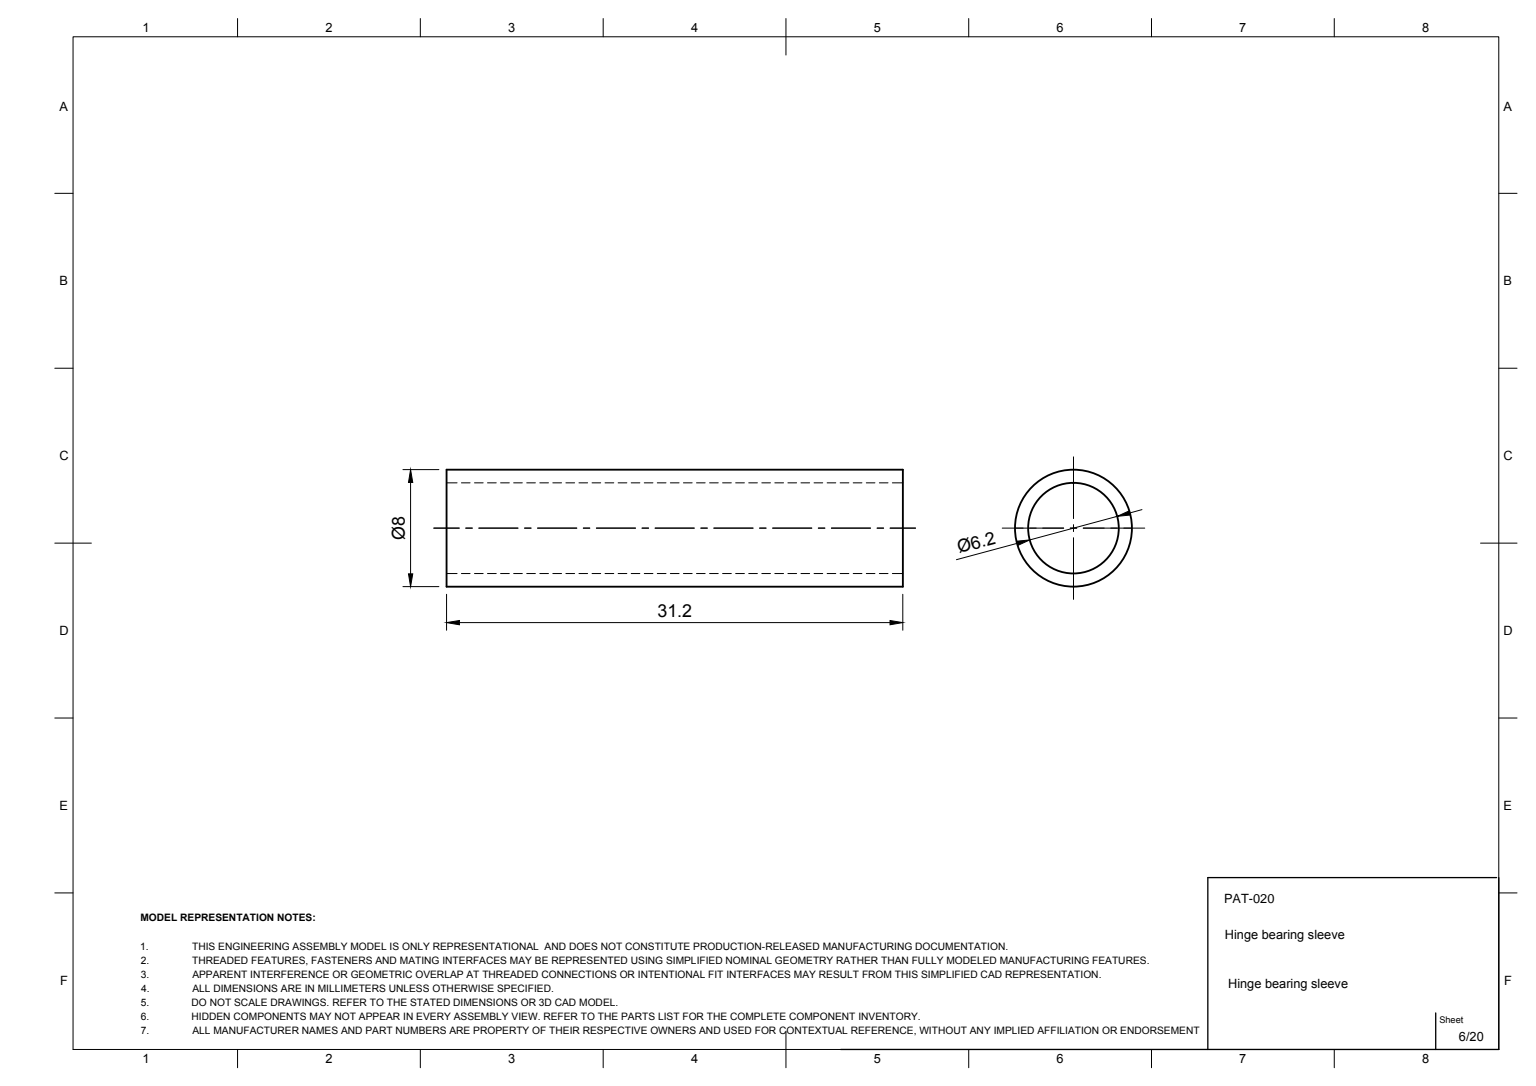
ISO-10303-21;
HEADER;
/* Generated by software containing ST-Developer
 * from STEP Tools, Inc. (www.steptools.com) 
 */

FILE_DESCRIPTION(
/* description */ ('Cable chain and bracket set'),
/* implementation_level */ '2;1');

FILE_NAME(
/* name */ 'Hinge bearing sleeve.step',
/* time_stamp */ '2026-10-29T17:19:47-07:00',
/* author */ (''),
/* organization */ (''),
/* preprocessor_version */ 'ST-DEVELOPER v20.2',
/* originating_system */ 'Autodesk Translation Framework v15.17.0.0',
/* authorisation */ '');

FILE_SCHEMA (('AUTOMOTIVE_DESIGN { 1 0 10303 214 3 1 1 }'));
ENDSEC;

DATA;
#10=MECHANICAL_DESIGN_GEOMETRIC_PRESENTATION_REPRESENTATION('',(#346),#5929);
#320=SHAPE_REPRESENTATION_RELATIONSHIP('SRR','None',#6058,#333);
#333=ADVANCED_BREP_SHAPE_REPRESENTATION('',(#359),#5925);
#346=STYLED_ITEM('',(#6220),#359);
#359=MANIFOLD_SOLID_BREP('Body1',#3340);
#397=FACE_BOUND('',#895,.T.);
#398=FACE_BOUND('',#897,.T.);
#505=PLANE('',#3714);
#506=PLANE('',#3715);
#676=FACE_OUTER_BOUND('',#892,.T.);
#677=FACE_OUTER_BOUND('',#893,.T.);
#678=FACE_OUTER_BOUND('',#894,.T.);
#679=FACE_OUTER_BOUND('',#896,.T.);
#892=EDGE_LOOP('',(#2967,#2968,#2969,#2970));
#893=EDGE_LOOP('',(#2971,#2972,#2973,#2974));
#894=EDGE_LOOP('',(#2975));
#895=EDGE_LOOP('',(#2976));
#896=EDGE_LOOP('',(#2977));
#897=EDGE_LOOP('',(#2978));
#1164=LINE('',#5655,#1424);
#1165=LINE('',#5661,#1425);
#1424=VECTOR('',#4621,0.31);
#1425=VECTOR('',#4628,0.4);
#1543=CIRCLE('',#3709,0.31);
#1544=CIRCLE('',#3710,0.31);
#1545=CIRCLE('',#3712,0.4);
#1546=CIRCLE('',#3713,0.4);
#1783=VERTEX_POINT('',#5652);
#1784=VERTEX_POINT('',#5654);
#1785=VERTEX_POINT('',#5658);
#1786=VERTEX_POINT('',#5660);
#2184=EDGE_CURVE('',#1783,#1783,#1543,.T.);
#2185=EDGE_CURVE('',#1783,#1784,#1164,.T.);
#2186=EDGE_CURVE('',#1784,#1784,#1544,.T.);
#2187=EDGE_CURVE('',#1785,#1785,#1545,.T.);
#2188=EDGE_CURVE('',#1785,#1786,#1165,.T.);
#2189=EDGE_CURVE('',#1786,#1786,#1546,.T.);
#2967=ORIENTED_EDGE('',*,*,#2184,.F.);
#2968=ORIENTED_EDGE('',*,*,#2185,.T.);
#2969=ORIENTED_EDGE('',*,*,#2186,.T.);
#2970=ORIENTED_EDGE('',*,*,#2185,.F.);
#2971=ORIENTED_EDGE('',*,*,#2187,.F.);
#2972=ORIENTED_EDGE('',*,*,#2188,.T.);
#2973=ORIENTED_EDGE('',*,*,#2189,.T.);
#2974=ORIENTED_EDGE('',*,*,#2188,.F.);
#2975=ORIENTED_EDGE('',*,*,#2187,.T.);
#2976=ORIENTED_EDGE('',*,*,#2184,.T.);
#2977=ORIENTED_EDGE('',*,*,#2189,.F.);
#2978=ORIENTED_EDGE('',*,*,#2186,.F.);
#3142=CYLINDRICAL_SURFACE('',#3708,0.31);
#3143=CYLINDRICAL_SURFACE('',#3711,0.4);
#3298=ADVANCED_FACE('',(#676),#3142,.F.);
#3299=ADVANCED_FACE('',(#677),#3143,.T.);
#3300=ADVANCED_FACE('',(#678,#397),#505,.T.);
#3301=ADVANCED_FACE('',(#679,#398),#506,.F.);
#3340=CLOSED_SHELL('',(#3298,#3299,#3300,#3301));
#3707=AXIS2_PLACEMENT_3D('',#5650,#4615,#4616);
#3708=AXIS2_PLACEMENT_3D('',#5651,#4617,#4618);
#3709=AXIS2_PLACEMENT_3D('',#5653,#4619,#4620);
#3710=AXIS2_PLACEMENT_3D('',#5656,#4622,#4623);
#3711=AXIS2_PLACEMENT_3D('',#5657,#4624,#4625);
#3712=AXIS2_PLACEMENT_3D('',#5659,#4626,#4627);
#3713=AXIS2_PLACEMENT_3D('',#5662,#4629,#4630);
#3714=AXIS2_PLACEMENT_3D('',#5663,#4631,#4632);
#3715=AXIS2_PLACEMENT_3D('',#5664,#4633,#4634);
#4615=DIRECTION('axis',(0.,0.,1.));
#4616=DIRECTION('refdir',(1.,0.,0.));
#4617=DIRECTION('center_axis',(0.,1.,0.));
#4618=DIRECTION('ref_axis',(1.,0.,0.));
#4619=DIRECTION('center_axis',(0.,-1.,0.));
#4620=DIRECTION('ref_axis',(1.,0.,0.));
#4621=DIRECTION('',(0.,-1.,0.));
#4622=DIRECTION('center_axis',(0.,-1.,0.));
#4623=DIRECTION('ref_axis',(1.,0.,0.));
#4624=DIRECTION('center_axis',(0.,1.,0.));
#4625=DIRECTION('ref_axis',(1.,0.,0.));
#4626=DIRECTION('center_axis',(0.,1.,0.));
#4627=DIRECTION('ref_axis',(1.,0.,0.));
#4628=DIRECTION('',(0.,-1.,0.));
#4629=DIRECTION('center_axis',(0.,1.,0.));
#4630=DIRECTION('ref_axis',(1.,0.,0.));
#4631=DIRECTION('center_axis',(0.,1.,0.));
#4632=DIRECTION('ref_axis',(1.,0.,0.));
#4633=DIRECTION('center_axis',(0.,1.,0.));
#4634=DIRECTION('ref_axis',(1.,0.,0.));
#5650=CARTESIAN_POINT('',(0.,0.,0.));
#5651=CARTESIAN_POINT('Origin',(0.,-1.56,3.));
#5652=CARTESIAN_POINT('',(-0.31,1.56,3.));
#5653=CARTESIAN_POINT('Origin',(0.,1.56,3.));
#5654=CARTESIAN_POINT('',(-0.31,-1.56,3.));
#5655=CARTESIAN_POINT('',(-0.31,-1.56,3.));
#5656=CARTESIAN_POINT('Origin',(0.,-1.56,3.));
#5657=CARTESIAN_POINT('Origin',(0.,-1.56,3.));
#5658=CARTESIAN_POINT('',(-0.4,1.56,3.));
#5659=CARTESIAN_POINT('Origin',(0.,1.56,3.));
#5660=CARTESIAN_POINT('',(-0.4,-1.56,3.));
#5661=CARTESIAN_POINT('',(-0.4,-1.56,3.));
#5662=CARTESIAN_POINT('Origin',(0.,-1.56,3.));
#5663=CARTESIAN_POINT('Origin',(0.,1.56,3.));
#5664=CARTESIAN_POINT('Origin',(0.,-1.56,3.));
#5901=UNCERTAINTY_MEASURE_WITH_UNIT(LENGTH_MEASURE(0.001),#5930,
'DISTANCE_ACCURACY_VALUE',
'Maximum model space distance between geometric entities at asserted c
onnectivities');
#5905=UNCERTAINTY_MEASURE_WITH_UNIT(LENGTH_MEASURE(0.001),#5930,
'DISTANCE_ACCURACY_VALUE',
'Maximum model space distance between geometric entities at asserted c
onnectivities');
#5925=(
GEOMETRIC_REPRESENTATION_CONTEXT(3)
GLOBAL_UNCERTAINTY_ASSIGNED_CONTEXT((#5901))
GLOBAL_UNIT_ASSIGNED_CONTEXT((#5930,#5932,#5933))
REPRESENTATION_CONTEXT('','3D')
);
#5929=(
GEOMETRIC_REPRESENTATION_CONTEXT(3)
GLOBAL_UNCERTAINTY_ASSIGNED_CONTEXT((#5905))
GLOBAL_UNIT_ASSIGNED_CONTEXT((#5930,#5932,#5933))
REPRESENTATION_CONTEXT('','3D')
);
#5930=(
LENGTH_UNIT()
NAMED_UNIT(*)
SI_UNIT(.CENTI.,.METRE.)
);
#5932=(
NAMED_UNIT(*)
PLANE_ANGLE_UNIT()
SI_UNIT($,.RADIAN.)
);
#5933=(
NAMED_UNIT(*)
SI_UNIT($,.STERADIAN.)
SOLID_ANGLE_UNIT()
);
#5953=SHAPE_DEFINITION_REPRESENTATION(#5983,#6058);
#5983=PRODUCT_DEFINITION_SHAPE('',$,#6082);
#6058=SHAPE_REPRESENTATION('',(#3707),#5925);
#6062=PRODUCT_DEFINITION_CONTEXT('part definition',#6133,'design');
#6082=PRODUCT_DEFINITION('Hinge bearing sleeve',
'Hinge bearing sleeve',#6105,#6062);
#6105=PRODUCT_DEFINITION_FORMATION('',$,#6154);
#6133=APPLICATION_CONTEXT(
'Core Data for Automotive Mechanical Design Process');
#6134=PRODUCT_CONTEXT('part definition',#6133,'mechanical');
#6154=PRODUCT('Hinge bearing sleeve','Hinge bearing sleeve',
'Hinge bearing sleeve',(#6134));
#6214=COLOUR_RGB('Grey',0.48,0.52,0.57);
#6215=FILL_AREA_STYLE_COLOUR('',#6214);
#6216=FILL_AREA_STYLE('',(#6215));
#6217=SURFACE_STYLE_FILL_AREA(#6216);
#6218=SURFACE_SIDE_STYLE('',(#6217));
#6219=SURFACE_STYLE_USAGE(.BOTH.,#6218);
#6220=PRESENTATION_STYLE_ASSIGNMENT((#6219));
ENDSEC;
END-ISO-10303-21;
